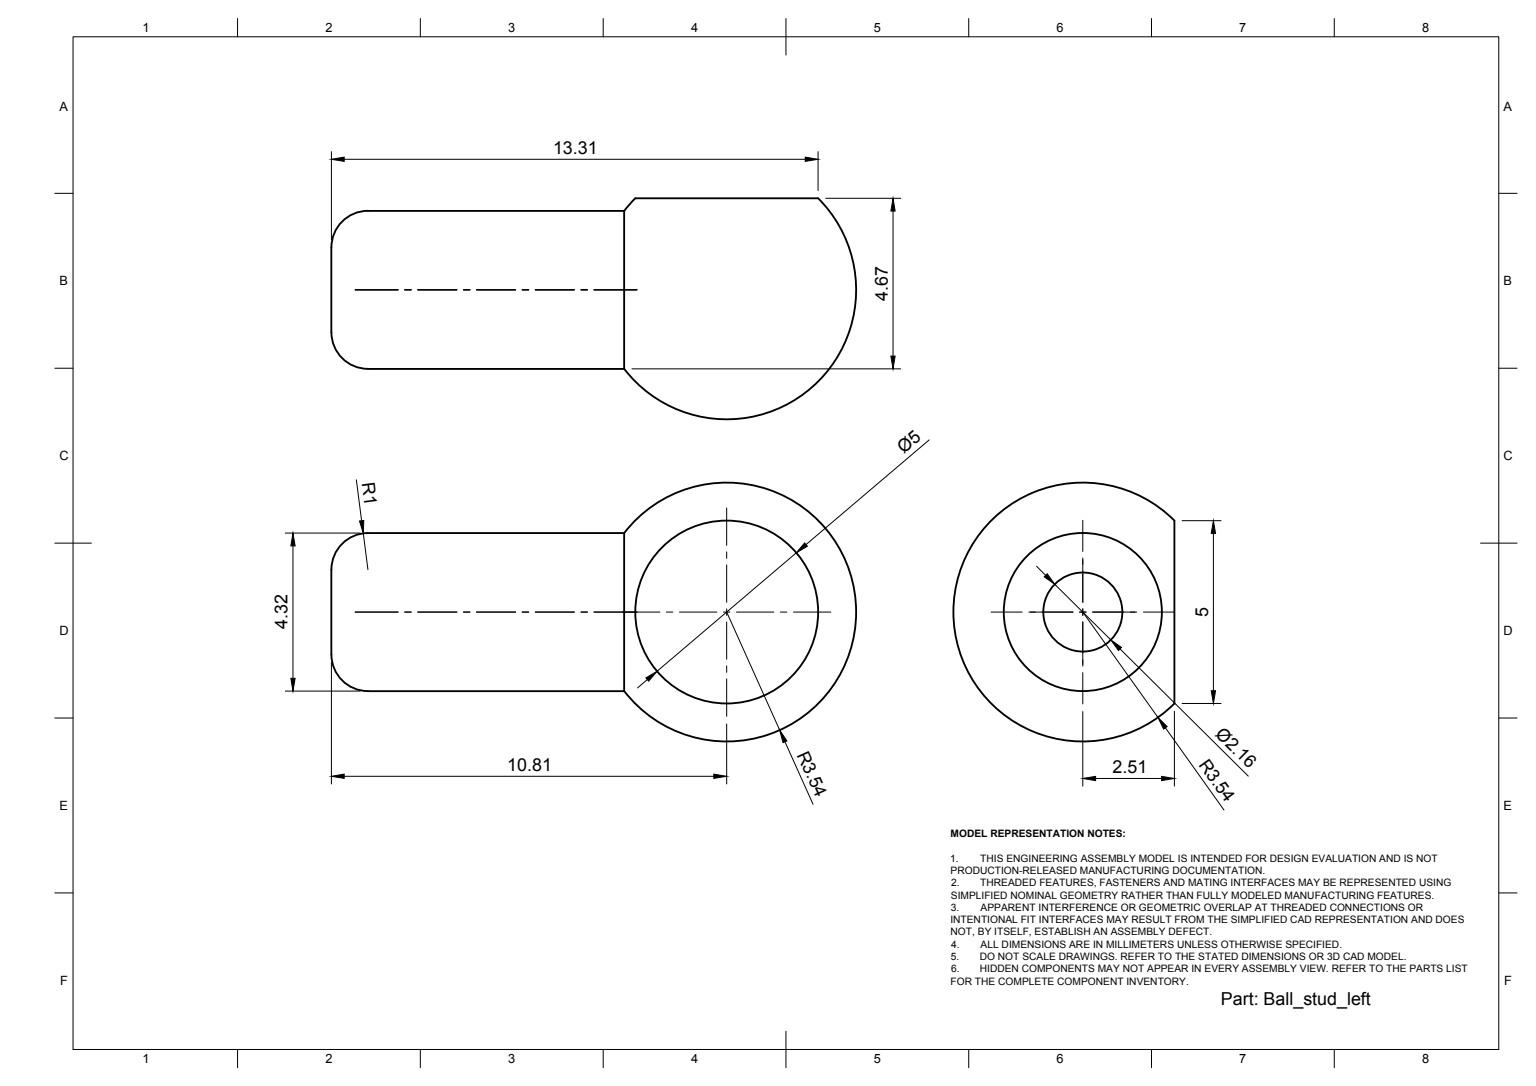
ISO-10303-21;
HEADER;
/* Generated by software containing ST-Developer
 * from STEP Tools, Inc. (www.steptools.com) 
 */

FILE_DESCRIPTION(
/* description */ (''),
/* implementation_level */ '2;1');

FILE_NAME(
/* name */ 'Ball_Stud_left.step',
/* time_stamp */ '2026-10-04T22:13:49-07:00',
/* author */ (''),
/* organization */ (''),
/* preprocessor_version */ 'ST-DEVELOPER v20.2',
/* originating_system */ 'Autodesk Translation Framework v15.15.0.0',
/* authorisation */ '');

FILE_SCHEMA (('AUTOMOTIVE_DESIGN { 1 0 10303 214 3 1 1 }'));
ENDSEC;

DATA;
#10=MECHANICAL_DESIGN_GEOMETRIC_PRESENTATION_REPRESENTATION('',(#361),#40734);
#345=SHAPE_REPRESENTATION_RELATIONSHIP('SRR','None',#40766,#353);
#353=ADVANCED_BREP_SHAPE_REPRESENTATION('',(#370),#40726);
#361=STYLED_ITEM('',(#40815),#370);
#370=MANIFOLD_SOLID_BREP('Body1',#3166);
#379=SPHERICAL_SURFACE('',#3282,3.53951905042299);
#381=FACE_BOUND('',#591,.T.);
#382=FACE_BOUND('',#596,.T.);
#391=TOROIDAL_SURFACE('',#3270,1.16126351211314,1.);
#395=PLANE('',#3269);
#396=PLANE('',#3274);
#397=PLANE('',#3281);
#427=FACE_OUTER_BOUND('',#587,.T.);
#428=FACE_OUTER_BOUND('',#588,.T.);
#429=FACE_OUTER_BOUND('',#589,.T.);
#430=FACE_OUTER_BOUND('',#590,.T.);
#431=FACE_OUTER_BOUND('',#592,.T.);
#432=FACE_OUTER_BOUND('',#593,.T.);
#433=FACE_OUTER_BOUND('',#594,.T.);
#434=FACE_OUTER_BOUND('',#595,.T.);
#587=EDGE_LOOP('',(#1922,#1923,#1924,#1925));
#588=EDGE_LOOP('',(#1926));
#589=EDGE_LOOP('',(#1927,#1928,#1929,#1930));
#590=EDGE_LOOP('',(#1931));
#591=EDGE_LOOP('',(#1932));
#592=EDGE_LOOP('',(#1933,#1934,#1935,#1936,#1937));
#593=EDGE_LOOP('',(#1938,#1939,#1940,#1941));
#594=EDGE_LOOP('',(#1942));
#595=EDGE_LOOP('',(#1943,#1944,#1945,#1946));
#596=EDGE_LOOP('',(#1947));
#757=LINE('',#4066,#899);
#758=LINE('',#4078,#900);
#759=LINE('',#4086,#901);
#899=VECTOR('',#3490,1.08063175605657);
#900=VECTOR('',#3507,2.16126351211314);
#901=VECTOR('',#3516,2.5);
#1041=CIRCLE('',#3267,1.08063175605657);
#1042=CIRCLE('',#3268,1.08063175605657);
#1043=CIRCLE('',#3271,1.16126351211314);
#1044=CIRCLE('',#3272,1.);
#1045=CIRCLE('',#3273,2.16126351211314);
#1046=CIRCLE('',#3276,2.16126351211314);
#1047=CIRCLE('',#3277,2.16126351211314);
#1048=CIRCLE('',#3279,2.5);
#1049=CIRCLE('',#3280,2.5);
#1050=CIRCLE('',#3283,3.53951905042299);
#1090=VERTEX_POINT('',#4063);
#1091=VERTEX_POINT('',#4065);
#1092=VERTEX_POINT('',#4070);
#1093=VERTEX_POINT('',#4072);
#1094=VERTEX_POINT('',#4077);
#1095=VERTEX_POINT('',#4079);
#1096=VERTEX_POINT('',#4083);
#1097=VERTEX_POINT('',#4085);
#1098=VERTEX_POINT('',#4090);
#1437=EDGE_CURVE('',#1090,#1090,#1041,.T.);
#1438=EDGE_CURVE('',#1090,#1091,#757,.T.);
#1439=EDGE_CURVE('',#1091,#1091,#1042,.T.);
#1440=EDGE_CURVE('',#1092,#1092,#1043,.T.);
#1441=EDGE_CURVE('',#1092,#1093,#1044,.T.);
#1442=EDGE_CURVE('',#1093,#1093,#1045,.T.);
#1443=EDGE_CURVE('',#1093,#1094,#758,.T.);
#1444=EDGE_CURVE('',#1094,#1095,#1046,.T.);
#1445=EDGE_CURVE('',#1095,#1094,#1047,.T.);
#1446=EDGE_CURVE('',#1096,#1096,#1048,.T.);
#1447=EDGE_CURVE('',#1096,#1097,#759,.T.);
#1448=EDGE_CURVE('',#1097,#1097,#1049,.T.);
#1449=EDGE_CURVE('',#1095,#1098,#1050,.T.);
#1922=ORIENTED_EDGE('',*,*,#1437,.F.);
#1923=ORIENTED_EDGE('',*,*,#1438,.T.);
#1924=ORIENTED_EDGE('',*,*,#1439,.T.);
#1925=ORIENTED_EDGE('',*,*,#1438,.F.);
#1926=ORIENTED_EDGE('',*,*,#1439,.F.);
#1927=ORIENTED_EDGE('',*,*,#1440,.T.);
#1928=ORIENTED_EDGE('',*,*,#1441,.T.);
#1929=ORIENTED_EDGE('',*,*,#1442,.T.);
#1930=ORIENTED_EDGE('',*,*,#1441,.F.);
#1931=ORIENTED_EDGE('',*,*,#1440,.F.);
#1932=ORIENTED_EDGE('',*,*,#1437,.T.);
#1933=ORIENTED_EDGE('',*,*,#1442,.F.);
#1934=ORIENTED_EDGE('',*,*,#1443,.T.);
#1935=ORIENTED_EDGE('',*,*,#1444,.T.);
#1936=ORIENTED_EDGE('',*,*,#1445,.T.);
#1937=ORIENTED_EDGE('',*,*,#1443,.F.);
#1938=ORIENTED_EDGE('',*,*,#1446,.T.);
#1939=ORIENTED_EDGE('',*,*,#1447,.T.);
#1940=ORIENTED_EDGE('',*,*,#1448,.F.);
#1941=ORIENTED_EDGE('',*,*,#1447,.F.);
#1942=ORIENTED_EDGE('',*,*,#1446,.F.);
#1943=ORIENTED_EDGE('',*,*,#1445,.F.);
#1944=ORIENTED_EDGE('',*,*,#1449,.T.);
#1945=ORIENTED_EDGE('',*,*,#1449,.F.);
#1946=ORIENTED_EDGE('',*,*,#1444,.F.);
#1947=ORIENTED_EDGE('',*,*,#1448,.T.);
#2892=CYLINDRICAL_SURFACE('',#3266,1.08063175605657);
#2893=CYLINDRICAL_SURFACE('',#3275,2.16126351211314);
#2894=CYLINDRICAL_SURFACE('',#3278,2.5);
#3006=ADVANCED_FACE('',(#427),#2892,.F.);
#3007=ADVANCED_FACE('',(#428),#395,.T.);
#3008=ADVANCED_FACE('',(#429),#391,.T.);
#3009=ADVANCED_FACE('',(#430,#381),#396,.T.);
#3010=ADVANCED_FACE('',(#431),#2893,.T.);
#3011=ADVANCED_FACE('',(#432),#2894,.F.);
#3012=ADVANCED_FACE('',(#433),#397,.F.);
#3013=ADVANCED_FACE('',(#434,#382),#379,.T.);
#3166=CLOSED_SHELL('',(#3006,#3007,#3008,#3009,#3010,#3011,#3012,#3013));
#3265=AXIS2_PLACEMENT_3D('',#4061,#3484,#3485);
#3266=AXIS2_PLACEMENT_3D('',#4062,#3486,#3487);
#3267=AXIS2_PLACEMENT_3D('',#4064,#3488,#3489);
#3268=AXIS2_PLACEMENT_3D('',#4067,#3491,#3492);
#3269=AXIS2_PLACEMENT_3D('',#4068,#3493,#3494);
#3270=AXIS2_PLACEMENT_3D('',#4069,#3495,#3496);
#3271=AXIS2_PLACEMENT_3D('',#4071,#3497,#3498);
#3272=AXIS2_PLACEMENT_3D('',#4073,#3499,#3500);
#3273=AXIS2_PLACEMENT_3D('',#4074,#3501,#3502);
#3274=AXIS2_PLACEMENT_3D('',#4075,#3503,#3504);
#3275=AXIS2_PLACEMENT_3D('',#4076,#3505,#3506);
#3276=AXIS2_PLACEMENT_3D('',#4080,#3508,#3509);
#3277=AXIS2_PLACEMENT_3D('',#4081,#3510,#3511);
#3278=AXIS2_PLACEMENT_3D('',#4082,#3512,#3513);
#3279=AXIS2_PLACEMENT_3D('',#4084,#3514,#3515);
#3280=AXIS2_PLACEMENT_3D('',#4087,#3517,#3518);
#3281=AXIS2_PLACEMENT_3D('',#4088,#3519,#3520);
#3282=AXIS2_PLACEMENT_3D('',#4089,#3521,#3522);
#3283=AXIS2_PLACEMENT_3D('',#4091,#3523,#3524);
#3484=DIRECTION('axis',(0.,0.,1.));
#3485=DIRECTION('refdir',(1.,0.,0.));
#3486=DIRECTION('center_axis',(-1.,0.,0.));
#3487=DIRECTION('ref_axis',(0.,1.,0.));
#3488=DIRECTION('center_axis',(-1.,0.,0.));
#3489=DIRECTION('ref_axis',(0.,1.,0.));
#3490=DIRECTION('',(-1.,0.,0.));
#3491=DIRECTION('center_axis',(-1.,0.,0.));
#3492=DIRECTION('ref_axis',(0.,1.,0.));
#3493=DIRECTION('center_axis',(1.,0.,0.));
#3494=DIRECTION('ref_axis',(0.,1.,0.));
#3495=DIRECTION('center_axis',(1.,0.,0.));
#3496=DIRECTION('ref_axis',(0.,0.,-1.));
#3497=DIRECTION('center_axis',(-1.,0.,0.));
#3498=DIRECTION('ref_axis',(0.,1.22464679914735E-16,1.));
#3499=DIRECTION('center_axis',(0.,-1.,-1.22464679914735E-16));
#3500=DIRECTION('ref_axis',(0.,-1.22464679914735E-16,1.));
#3501=DIRECTION('center_axis',(1.,0.,0.));
#3502=DIRECTION('ref_axis',(0.,1.22464679914735E-16,1.));
#3503=DIRECTION('center_axis',(1.,0.,0.));
#3504=DIRECTION('ref_axis',(0.,0.,-1.));
#3505=DIRECTION('center_axis',(1.,0.,0.));
#3506=DIRECTION('ref_axis',(0.,0.,-1.));
#3507=DIRECTION('',(-1.,0.,0.));
#3508=DIRECTION('center_axis',(1.,0.,0.));
#3509=DIRECTION('ref_axis',(0.,0.,-1.));
#3510=DIRECTION('center_axis',(1.,0.,0.));
#3511=DIRECTION('ref_axis',(0.,0.,-1.));
#3512=DIRECTION('center_axis',(0.,0.,-1.));
#3513=DIRECTION('ref_axis',(1.,0.,0.));
#3514=DIRECTION('center_axis',(0.,0.,1.));
#3515=DIRECTION('ref_axis',(1.,0.,0.));
#3516=DIRECTION('',(0.,0.,-1.));
#3517=DIRECTION('center_axis',(0.,0.,1.));
#3518=DIRECTION('ref_axis',(1.,0.,0.));
#3519=DIRECTION('center_axis',(0.,0.,1.));
#3520=DIRECTION('ref_axis',(1.,0.,0.));
#3521=DIRECTION('center_axis',(1.,-1.22464679914735E-16,0.));
#3522=DIRECTION('ref_axis',(0.,-1.,0.));
#3523=DIRECTION('center_axis',(-7.49879891330929E-33,-1.22464679914735E-16,
1.));
#3524=DIRECTION('ref_axis',(0.,1.,1.22464679914735E-16));
#4061=CARTESIAN_POINT('',(0.,0.,0.));
#4062=CARTESIAN_POINT('Origin',(67.3063659679149,0.,0.));
#4063=CARTESIAN_POINT('',(14.3512997641764,-1.08063175605657,1.32339222111166E-16));
#4064=CARTESIAN_POINT('Origin',(14.3512997641764,0.,0.));
#4065=CARTESIAN_POINT('',(9.05579314380255,-1.08063175605657,-1.32339222111166E-16));
#4066=CARTESIAN_POINT('',(67.3063659679149,-1.08063175605657,1.32339222111166E-16));
#4067=CARTESIAN_POINT('Origin',(9.05579314380255,0.,0.));
#4068=CARTESIAN_POINT('Origin',(9.05579314380255,0.,0.));
#4069=CARTESIAN_POINT('Origin',(13.3512997641764,0.,0.));
#4070=CARTESIAN_POINT('',(14.3512997641764,-1.42213764307597E-16,1.16126351211314));
#4071=CARTESIAN_POINT('Origin',(14.3512997641764,0.,0.));
#4072=CARTESIAN_POINT('',(13.3512997641764,-2.64678444222332E-16,2.16126351211314));
#4073=CARTESIAN_POINT('Origin',(13.3512997641764,-1.42213764307597E-16,
1.16126351211314));
#4074=CARTESIAN_POINT('Origin',(13.3512997641764,0.,0.));
#4075=CARTESIAN_POINT('Origin',(14.3512997641764,0.,0.));
#4076=CARTESIAN_POINT('Origin',(10.3469384954313,0.,0.));
#4077=CARTESIAN_POINT('',(6.34257722668614,-2.64678444222332E-16,2.16126351211314));
#4078=CARTESIAN_POINT('',(10.3469384954313,-2.64678444222332E-16,2.16126351211314));
#4079=CARTESIAN_POINT('',(6.34257722668614,2.16126351211314,2.64678444222332E-16));
#4080=CARTESIAN_POINT('Origin',(6.34257722668614,0.,0.));
#4081=CARTESIAN_POINT('Origin',(6.34257722668614,0.,0.));
#4082=CARTESIAN_POINT('Origin',(3.53951905042299,8.32667268468867E-16,0.));
#4083=CARTESIAN_POINT('',(1.03951905042299,5.26505568682029E-16,0.));
#4084=CARTESIAN_POINT('Origin',(3.53951905042299,8.32667268468867E-16,0.));
#4085=CARTESIAN_POINT('',(1.03951905042299,5.26505568682029E-16,-2.5056326762531));
#4086=CARTESIAN_POINT('',(1.03951905042299,1.13882896825571E-15,0.));
#4087=CARTESIAN_POINT('Origin',(3.53951905042299,8.32667268468867E-16,-2.5056326762531));
#4088=CARTESIAN_POINT('Origin',(3.53951905042299,6.93889390390723E-16,0.));
#4089=CARTESIAN_POINT('Origin',(3.53951905042299,0.,0.));
#4090=CARTESIAN_POINT('',(0.,2.1673303378108E-16,-1.3684555315672E-47));
#4091=CARTESIAN_POINT('Origin',(3.53951905042299,0.,0.));
#40716=UNCERTAINTY_MEASURE_WITH_UNIT(LENGTH_MEASURE(0.01),#40735,
'DISTANCE_ACCURACY_VALUE',
'Maximum model space distance between geometric entities at asserted c
onnectivities');
#40724=UNCERTAINTY_MEASURE_WITH_UNIT(LENGTH_MEASURE(0.01),#40735,
'DISTANCE_ACCURACY_VALUE',
'Maximum model space distance between geometric entities at asserted c
onnectivities');
#40726=(
GEOMETRIC_REPRESENTATION_CONTEXT(3)
GLOBAL_UNCERTAINTY_ASSIGNED_CONTEXT((#40716))
GLOBAL_UNIT_ASSIGNED_CONTEXT((#40735,#40737,#40738))
REPRESENTATION_CONTEXT('','3D')
);
#40734=(
GEOMETRIC_REPRESENTATION_CONTEXT(3)
GLOBAL_UNCERTAINTY_ASSIGNED_CONTEXT((#40724))
GLOBAL_UNIT_ASSIGNED_CONTEXT((#40735,#40737,#40738))
REPRESENTATION_CONTEXT('','3D')
);
#40735=(
LENGTH_UNIT()
NAMED_UNIT(*)
SI_UNIT(.MILLI.,.METRE.)
);
#40737=(
NAMED_UNIT(*)
PLANE_ANGLE_UNIT()
SI_UNIT($,.RADIAN.)
);
#40738=(
NAMED_UNIT(*)
SI_UNIT($,.STERADIAN.)
SOLID_ANGLE_UNIT()
);
#40740=SHAPE_DEFINITION_REPRESENTATION(#40749,#40766);
#40749=PRODUCT_DEFINITION_SHAPE('',$,#40776);
#40766=SHAPE_REPRESENTATION('',(#3265),#40726);
#40774=PRODUCT_DEFINITION_CONTEXT('part definition',#40803,'design');
#40776=PRODUCT_DEFINITION('Ball_Stud','Ball_Stud_left',#40785,#40774);
#40785=PRODUCT_DEFINITION_FORMATION('',$,#40806);
#40803=APPLICATION_CONTEXT(
'Core Data for Automotive Mechanical Design Process');
#40804=PRODUCT_CONTEXT('part definition',#40803,'mechanical');
#40806=PRODUCT('Ball_Stud','Ball_Stud_left',$,(#40804));
#40815=PRESENTATION_STYLE_ASSIGNMENT((#40818));
#40818=SURFACE_STYLE_USAGE(.BOTH.,#40821);
#40821=SURFACE_SIDE_STYLE('',(#40824));
#40824=SURFACE_STYLE_FILL_AREA(#40827);
#40827=FILL_AREA_STYLE('Opaque(203,203,203)',(#40830));
#40830=FILL_AREA_STYLE_COLOUR('Opaque(203,203,203)',#40833);
#40833=COLOUR_RGB('Opaque(203,203,203)', 0.09019608, 0.27058824, 0.51372549);
ENDSEC;
END-ISO-10303-21;
